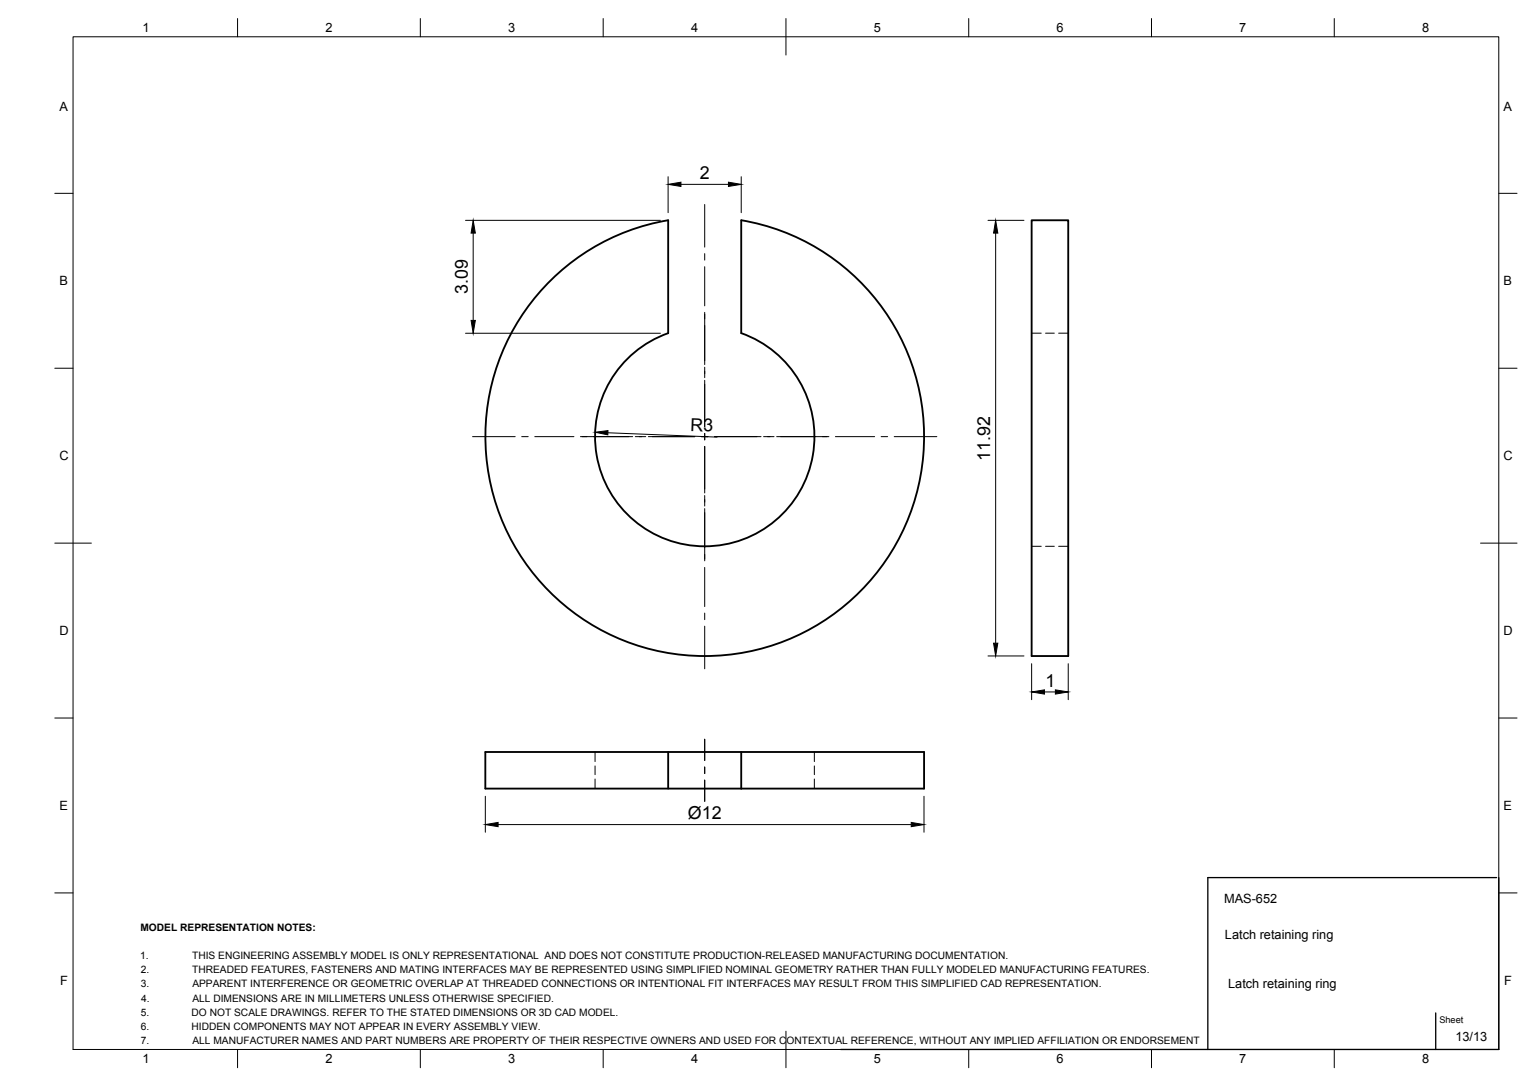
ISO-10303-21;
HEADER;
/* Generated by software containing ST-Developer
 * from STEP Tools, Inc. (www.steptools.com) 
 */

FILE_DESCRIPTION(
/* description */ ('Independent hinged machine back cover with retained hinge pins, perim
eter gasket and quarter-turn cam latch. Nominal cover 360 x 260 x 3 mm
, frame 430 x 300 x 20 mm. No guarding, structural or ingress rating a
ssigned.'),
/* implementation_level */ '2;1');

FILE_NAME(
/* name */ 'Latch retaining ring.step',
/* time_stamp */ '2026-11-09T19:36:59-08:00',
/* author */ (''),
/* organization */ (''),
/* preprocessor_version */ 'ST-DEVELOPER v20.2',
/* originating_system */ 'Autodesk Translation Framework v15.17.0.0',
/* authorisation */ '');

FILE_SCHEMA (('AUTOMOTIVE_DESIGN { 1 0 10303 214 3 1 1 }'));
ENDSEC;

DATA;
#10=MECHANICAL_DESIGN_GEOMETRIC_PRESENTATION_REPRESENTATION('',(#204),#32627);
#168=SHAPE_REPRESENTATION_RELATIONSHIP('SRR','None',#32714,#186);
#186=ADVANCED_BREP_SHAPE_REPRESENTATION('',(#222),#32615);
#204=STYLED_ITEM('',(#32809),#222);
#222=MANIFOLD_SOLID_BREP('Body1',#8681);
#378=PLANE('',#9206);
#379=PLANE('',#9207);
#380=PLANE('',#9208);
#381=PLANE('',#9215);
#717=FACE_OUTER_BOUND('',#1220,.T.);
#718=FACE_OUTER_BOUND('',#1221,.T.);
#719=FACE_OUTER_BOUND('',#1222,.T.);
#720=FACE_OUTER_BOUND('',#1223,.T.);
#721=FACE_OUTER_BOUND('',#1224,.T.);
#722=FACE_OUTER_BOUND('',#1225,.T.);
#1220=EDGE_LOOP('',(#6825,#6826,#6827,#6828));
#1221=EDGE_LOOP('',(#6829,#6830,#6831,#6832));
#1222=EDGE_LOOP('',(#6833,#6834,#6835,#6836));
#1223=EDGE_LOOP('',(#6837,#6838,#6839,#6840));
#1224=EDGE_LOOP('',(#6841,#6842,#6843,#6844));
#1225=EDGE_LOOP('',(#6845,#6846,#6847,#6848));
#1512=CIRCLE('',#9209,6.);
#1513=CIRCLE('',#9210,3.);
#1514=CIRCLE('',#9212,3.);
#1515=CIRCLE('',#9214,6.);
#2478=LINE('',#24284,#3024);
#2479=LINE('',#24286,#3025);
#2480=LINE('',#24288,#3026);
#2481=LINE('',#24289,#3027);
#2482=LINE('',#24293,#3028);
#2483=LINE('',#24295,#3029);
#2484=LINE('',#24297,#3030);
#2485=LINE('',#24298,#3031);
#3024=VECTOR('',#10462,10.);
#3025=VECTOR('',#10463,10.);
#3026=VECTOR('',#10464,10.);
#3027=VECTOR('',#10465,10.);
#3028=VECTOR('',#10468,10.);
#3029=VECTOR('',#10469,10.);
#3030=VECTOR('',#10470,10.);
#3031=VECTOR('',#10471,10.);
#3753=VERTEX_POINT('',#24282);
#3754=VERTEX_POINT('',#24283);
#3755=VERTEX_POINT('',#24285);
#3756=VERTEX_POINT('',#24287);
#3757=VERTEX_POINT('',#24291);
#3758=VERTEX_POINT('',#24292);
#3759=VERTEX_POINT('',#24294);
#3760=VERTEX_POINT('',#24296);
#4836=EDGE_CURVE('',#3753,#3754,#2478,.T.);
#4837=EDGE_CURVE('',#3755,#3753,#2479,.T.);
#4838=EDGE_CURVE('',#3756,#3755,#2480,.T.);
#4839=EDGE_CURVE('',#3754,#3756,#2481,.T.);
#4840=EDGE_CURVE('',#3757,#3758,#2482,.T.);
#4841=EDGE_CURVE('',#3759,#3757,#2483,.T.);
#4842=EDGE_CURVE('',#3760,#3759,#2484,.T.);
#4843=EDGE_CURVE('',#3758,#3760,#2485,.T.);
#4844=EDGE_CURVE('',#3755,#3760,#1512,.T.);
#4845=EDGE_CURVE('',#3758,#3753,#1513,.T.);
#4846=EDGE_CURVE('',#3757,#3754,#1514,.T.);
#4847=EDGE_CURVE('',#3756,#3759,#1515,.T.);
#6825=ORIENTED_EDGE('',*,*,#4836,.F.);
#6826=ORIENTED_EDGE('',*,*,#4837,.F.);
#6827=ORIENTED_EDGE('',*,*,#4838,.F.);
#6828=ORIENTED_EDGE('',*,*,#4839,.F.);
#6829=ORIENTED_EDGE('',*,*,#4840,.F.);
#6830=ORIENTED_EDGE('',*,*,#4841,.F.);
#6831=ORIENTED_EDGE('',*,*,#4842,.F.);
#6832=ORIENTED_EDGE('',*,*,#4843,.F.);
#6833=ORIENTED_EDGE('',*,*,#4843,.T.);
#6834=ORIENTED_EDGE('',*,*,#4844,.F.);
#6835=ORIENTED_EDGE('',*,*,#4837,.T.);
#6836=ORIENTED_EDGE('',*,*,#4845,.F.);
#6837=ORIENTED_EDGE('',*,*,#4840,.T.);
#6838=ORIENTED_EDGE('',*,*,#4845,.T.);
#6839=ORIENTED_EDGE('',*,*,#4836,.T.);
#6840=ORIENTED_EDGE('',*,*,#4846,.F.);
#6841=ORIENTED_EDGE('',*,*,#4842,.T.);
#6842=ORIENTED_EDGE('',*,*,#4847,.F.);
#6843=ORIENTED_EDGE('',*,*,#4838,.T.);
#6844=ORIENTED_EDGE('',*,*,#4844,.T.);
#6845=ORIENTED_EDGE('',*,*,#4841,.T.);
#6846=ORIENTED_EDGE('',*,*,#4846,.T.);
#6847=ORIENTED_EDGE('',*,*,#4839,.T.);
#6848=ORIENTED_EDGE('',*,*,#4847,.T.);
#8075=CYLINDRICAL_SURFACE('',#9211,3.);
#8076=CYLINDRICAL_SURFACE('',#9213,6.);
#8465=ADVANCED_FACE('',(#717),#378,.F.);
#8466=ADVANCED_FACE('',(#718),#379,.F.);
#8467=ADVANCED_FACE('',(#719),#380,.F.);
#8468=ADVANCED_FACE('',(#720),#8075,.F.);
#8469=ADVANCED_FACE('',(#721),#8076,.T.);
#8470=ADVANCED_FACE('',(#722),#381,.T.);
#8681=CLOSED_SHELL('',(#8465,#8466,#8467,#8468,#8469,#8470));
#9205=AXIS2_PLACEMENT_3D('',#24280,#10458,#10459);
#9206=AXIS2_PLACEMENT_3D('',#24281,#10460,#10461);
#9207=AXIS2_PLACEMENT_3D('',#24290,#10466,#10467);
#9208=AXIS2_PLACEMENT_3D('',#24299,#10472,#10473);
#9209=AXIS2_PLACEMENT_3D('',#24300,#10474,#10475);
#9210=AXIS2_PLACEMENT_3D('',#24301,#10476,#10477);
#9211=AXIS2_PLACEMENT_3D('',#24302,#10478,#10479);
#9212=AXIS2_PLACEMENT_3D('',#24303,#10480,#10481);
#9213=AXIS2_PLACEMENT_3D('',#24304,#10482,#10483);
#9214=AXIS2_PLACEMENT_3D('',#24305,#10484,#10485);
#9215=AXIS2_PLACEMENT_3D('',#24306,#10486,#10487);
#10458=DIRECTION('axis',(0.,0.,1.));
#10459=DIRECTION('refdir',(1.,0.,0.));
#10460=DIRECTION('center_axis',(-1.,0.,0.));
#10461=DIRECTION('ref_axis',(0.,1.,0.));
#10462=DIRECTION('',(0.,0.,1.));
#10463=DIRECTION('',(0.,-1.,0.));
#10464=DIRECTION('',(0.,0.,-1.));
#10465=DIRECTION('',(0.,1.,0.));
#10466=DIRECTION('center_axis',(1.,0.,0.));
#10467=DIRECTION('ref_axis',(0.,-1.,0.));
#10468=DIRECTION('',(0.,0.,-1.));
#10469=DIRECTION('',(0.,-1.,0.));
#10470=DIRECTION('',(0.,0.,1.));
#10471=DIRECTION('',(0.,1.,0.));
#10472=DIRECTION('center_axis',(0.,0.,1.));
#10473=DIRECTION('ref_axis',(1.,0.,0.));
#10474=DIRECTION('center_axis',(0.,0.,1.));
#10475=DIRECTION('ref_axis',(1.,0.,0.));
#10476=DIRECTION('center_axis',(0.,0.,-1.));
#10477=DIRECTION('ref_axis',(1.,0.,0.));
#10478=DIRECTION('center_axis',(0.,0.,1.));
#10479=DIRECTION('ref_axis',(6.12323399573677E-17,-1.,0.));
#10480=DIRECTION('center_axis',(0.,0.,-1.));
#10481=DIRECTION('ref_axis',(1.,0.,0.));
#10482=DIRECTION('center_axis',(0.,0.,1.));
#10483=DIRECTION('ref_axis',(6.12323399573677E-17,-1.,0.));
#10484=DIRECTION('center_axis',(0.,0.,1.));
#10485=DIRECTION('ref_axis',(1.,0.,0.));
#10486=DIRECTION('center_axis',(0.,0.,1.));
#10487=DIRECTION('ref_axis',(1.,0.,0.));
#24280=CARTESIAN_POINT('',(0.,0.,0.));
#24281=CARTESIAN_POINT('Origin',(-1.,0.,1.));
#24282=CARTESIAN_POINT('',(-1.,2.82842712474619,0.));
#24283=CARTESIAN_POINT('',(-1.,2.82842712474619,1.));
#24284=CARTESIAN_POINT('',(-1.,2.82842712474619,0.));
#24285=CARTESIAN_POINT('',(-1.,5.91607978309962,0.));
#24286=CARTESIAN_POINT('',(-1.,0.,0.));
#24287=CARTESIAN_POINT('',(-1.,5.91607978309962,1.));
#24288=CARTESIAN_POINT('',(-1.,5.91607978309962,0.));
#24289=CARTESIAN_POINT('',(-1.,0.,1.));
#24290=CARTESIAN_POINT('Origin',(1.,12.,1.));
#24291=CARTESIAN_POINT('',(1.,2.82842712474619,1.));
#24292=CARTESIAN_POINT('',(1.,2.82842712474619,0.));
#24293=CARTESIAN_POINT('',(1.,2.82842712474619,0.));
#24294=CARTESIAN_POINT('',(1.,5.91607978309962,1.));
#24295=CARTESIAN_POINT('',(1.,6.,1.));
#24296=CARTESIAN_POINT('',(1.,5.91607978309962,0.));
#24297=CARTESIAN_POINT('',(1.,5.91607978309962,0.));
#24298=CARTESIAN_POINT('',(1.,6.,0.));
#24299=CARTESIAN_POINT('Origin',(0.,0.,0.));
#24300=CARTESIAN_POINT('Origin',(0.,0.,0.));
#24301=CARTESIAN_POINT('Origin',(0.,0.,0.));
#24302=CARTESIAN_POINT('Origin',(0.,0.,0.));
#24303=CARTESIAN_POINT('Origin',(0.,0.,1.));
#24304=CARTESIAN_POINT('Origin',(0.,0.,0.));
#24305=CARTESIAN_POINT('Origin',(0.,0.,1.));
#24306=CARTESIAN_POINT('Origin',(0.,0.,1.));
#32595=UNCERTAINTY_MEASURE_WITH_UNIT(LENGTH_MEASURE(0.01),#32628,
'DISTANCE_ACCURACY_VALUE',
'Maximum model space distance between geometric entities at asserted c
onnectivities');
#32607=UNCERTAINTY_MEASURE_WITH_UNIT(LENGTH_MEASURE(0.01),#32628,
'DISTANCE_ACCURACY_VALUE',
'Maximum model space distance between geometric entities at asserted c
onnectivities');
#32615=(
GEOMETRIC_REPRESENTATION_CONTEXT(3)
GLOBAL_UNCERTAINTY_ASSIGNED_CONTEXT((#32595))
GLOBAL_UNIT_ASSIGNED_CONTEXT((#32628,#32630,#32631))
REPRESENTATION_CONTEXT('','3D')
);
#32627=(
GEOMETRIC_REPRESENTATION_CONTEXT(3)
GLOBAL_UNCERTAINTY_ASSIGNED_CONTEXT((#32607))
GLOBAL_UNIT_ASSIGNED_CONTEXT((#32628,#32630,#32631))
REPRESENTATION_CONTEXT('','3D')
);
#32628=(
LENGTH_UNIT()
NAMED_UNIT(*)
SI_UNIT(.MILLI.,.METRE.)
);
#32630=(
NAMED_UNIT(*)
PLANE_ANGLE_UNIT()
SI_UNIT($,.RADIAN.)
);
#32631=(
NAMED_UNIT(*)
SI_UNIT($,.STERADIAN.)
SOLID_ANGLE_UNIT()
);
#32639=SHAPE_DEFINITION_REPRESENTATION(#32658,#32714);
#32658=PRODUCT_DEFINITION_SHAPE('',$,#32734);
#32714=SHAPE_REPRESENTATION('',(#9205),#32615);
#32726=PRODUCT_DEFINITION_CONTEXT('part definition',#32785,'design');
#32734=PRODUCT_DEFINITION('Latch retaining ring','Latch retaining ring',
#32753,#32726);
#32753=PRODUCT_DEFINITION_FORMATION('',$,#32794);
#32785=APPLICATION_CONTEXT(
'Core Data for Automotive Mechanical Design Process');
#32786=PRODUCT_CONTEXT('part definition',#32785,'mechanical');
#32794=PRODUCT('Latch retaining ring','Latch retaining ring',$,(#32786));
#32809=PRESENTATION_STYLE_ASSIGNMENT((#32816));
#32816=SURFACE_STYLE_USAGE(.BOTH.,#32823);
#32823=SURFACE_SIDE_STYLE('',(#32830));
#32830=SURFACE_STYLE_FILL_AREA(#32837);
#32837=FILL_AREA_STYLE('Dark gray',(#32844));
#32844=FILL_AREA_STYLE_COLOUR('Dark gray',#32851);
#32851=COLOUR_RGB('Dark gray',0.250980392156863,0.282352941176471,0.32156862745098);
ENDSEC;
END-ISO-10303-21;
